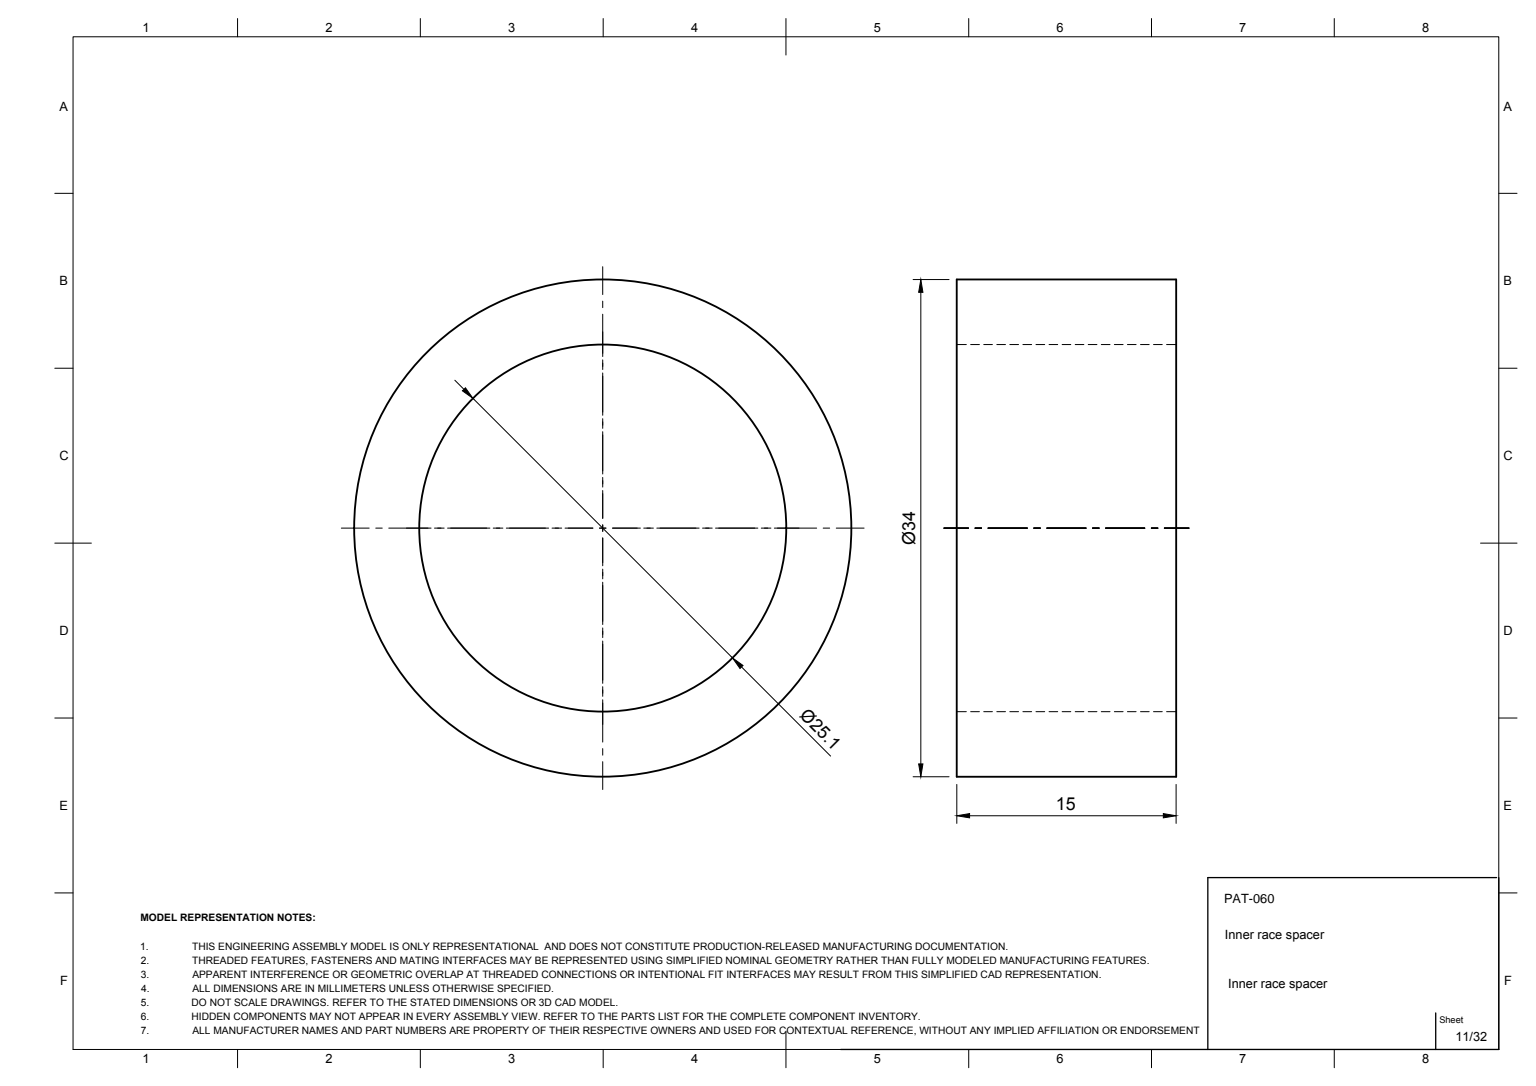
ISO-10303-21;
HEADER;
/* Generated by software containing ST-Developer
 * from STEP Tools, Inc. (www.steptools.com) 
 */

FILE_DESCRIPTION(
/* description */ ('Indexing fixture plate with plunger'),
/* implementation_level */ '2;1');

FILE_NAME(
/* name */ 'Inner race spacer.step',
/* time_stamp */ '2026-10-28T03:23:41-07:00',
/* author */ (''),
/* organization */ (''),
/* preprocessor_version */ 'ST-DEVELOPER v20.2',
/* originating_system */ 'Autodesk Translation Framework v15.17.0.0',
/* authorisation */ '');

FILE_SCHEMA (('AUTOMOTIVE_DESIGN { 1 0 10303 214 3 1 1 }'));
ENDSEC;

DATA;
#10=MECHANICAL_DESIGN_GEOMETRIC_PRESENTATION_REPRESENTATION('',(#323),#10020);
#269=SHAPE_REPRESENTATION_RELATIONSHIP('SRR','None',#10143,#296);
#296=ADVANCED_BREP_SHAPE_REPRESENTATION('',(#359),#9996);
#323=STYLED_ITEM('',(#10368),#359);
#359=MANIFOLD_SOLID_BREP('Body1',#4577);
#412=FACE_BOUND('',#1022,.T.);
#413=FACE_BOUND('',#1024,.T.);
#556=PLANE('',#4998);
#557=PLANE('',#4999);
#708=FACE_OUTER_BOUND('',#1019,.T.);
#709=FACE_OUTER_BOUND('',#1020,.T.);
#710=FACE_OUTER_BOUND('',#1021,.T.);
#711=FACE_OUTER_BOUND('',#1023,.T.);
#1019=EDGE_LOOP('',(#3201,#3202,#3203,#3204));
#1020=EDGE_LOOP('',(#3205,#3206,#3207,#3208));
#1021=EDGE_LOOP('',(#3209));
#1022=EDGE_LOOP('',(#3210));
#1023=EDGE_LOOP('',(#3211));
#1024=EDGE_LOOP('',(#3212));
#1423=LINE('',#7291,#1643);
#1424=LINE('',#7297,#1644);
#1643=VECTOR('',#5778,1.255);
#1644=VECTOR('',#5785,1.7);
#1870=CIRCLE('',#4993,1.255);
#1871=CIRCLE('',#4994,1.255);
#1872=CIRCLE('',#4996,1.7);
#1873=CIRCLE('',#4997,1.7);
#2181=VERTEX_POINT('',#7288);
#2182=VERTEX_POINT('',#7290);
#2183=VERTEX_POINT('',#7294);
#2184=VERTEX_POINT('',#7296);
#2580=EDGE_CURVE('',#2181,#2181,#1870,.T.);
#2581=EDGE_CURVE('',#2181,#2182,#1423,.T.);
#2582=EDGE_CURVE('',#2182,#2182,#1871,.T.);
#2583=EDGE_CURVE('',#2183,#2183,#1872,.T.);
#2584=EDGE_CURVE('',#2183,#2184,#1424,.T.);
#2585=EDGE_CURVE('',#2184,#2184,#1873,.T.);
#3201=ORIENTED_EDGE('',*,*,#2580,.F.);
#3202=ORIENTED_EDGE('',*,*,#2581,.T.);
#3203=ORIENTED_EDGE('',*,*,#2582,.T.);
#3204=ORIENTED_EDGE('',*,*,#2581,.F.);
#3205=ORIENTED_EDGE('',*,*,#2583,.F.);
#3206=ORIENTED_EDGE('',*,*,#2584,.T.);
#3207=ORIENTED_EDGE('',*,*,#2585,.T.);
#3208=ORIENTED_EDGE('',*,*,#2584,.F.);
#3209=ORIENTED_EDGE('',*,*,#2583,.T.);
#3210=ORIENTED_EDGE('',*,*,#2580,.T.);
#3211=ORIENTED_EDGE('',*,*,#2585,.F.);
#3212=ORIENTED_EDGE('',*,*,#2582,.F.);
#4186=CYLINDRICAL_SURFACE('',#4992,1.255);
#4187=CYLINDRICAL_SURFACE('',#4995,1.7);
#4323=ADVANCED_FACE('',(#708),#4186,.F.);
#4324=ADVANCED_FACE('',(#709),#4187,.T.);
#4325=ADVANCED_FACE('',(#710,#412),#556,.T.);
#4326=ADVANCED_FACE('',(#711,#413),#557,.F.);
#4577=CLOSED_SHELL('',(#4323,#4324,#4325,#4326));
#4991=AXIS2_PLACEMENT_3D('',#7286,#5772,#5773);
#4992=AXIS2_PLACEMENT_3D('',#7287,#5774,#5775);
#4993=AXIS2_PLACEMENT_3D('',#7289,#5776,#5777);
#4994=AXIS2_PLACEMENT_3D('',#7292,#5779,#5780);
#4995=AXIS2_PLACEMENT_3D('',#7293,#5781,#5782);
#4996=AXIS2_PLACEMENT_3D('',#7295,#5783,#5784);
#4997=AXIS2_PLACEMENT_3D('',#7298,#5786,#5787);
#4998=AXIS2_PLACEMENT_3D('',#7299,#5788,#5789);
#4999=AXIS2_PLACEMENT_3D('',#7300,#5790,#5791);
#5772=DIRECTION('axis',(0.,0.,1.));
#5773=DIRECTION('refdir',(1.,0.,0.));
#5774=DIRECTION('center_axis',(0.,0.,1.));
#5775=DIRECTION('ref_axis',(1.,0.,0.));
#5776=DIRECTION('center_axis',(0.,0.,-1.));
#5777=DIRECTION('ref_axis',(1.,0.,0.));
#5778=DIRECTION('',(0.,0.,-1.));
#5779=DIRECTION('center_axis',(0.,0.,-1.));
#5780=DIRECTION('ref_axis',(1.,0.,0.));
#5781=DIRECTION('center_axis',(0.,0.,1.));
#5782=DIRECTION('ref_axis',(1.,0.,0.));
#5783=DIRECTION('center_axis',(0.,0.,1.));
#5784=DIRECTION('ref_axis',(1.,0.,0.));
#5785=DIRECTION('',(0.,0.,-1.));
#5786=DIRECTION('center_axis',(0.,0.,1.));
#5787=DIRECTION('ref_axis',(1.,0.,0.));
#5788=DIRECTION('center_axis',(0.,0.,1.));
#5789=DIRECTION('ref_axis',(1.,0.,0.));
#5790=DIRECTION('center_axis',(0.,0.,1.));
#5791=DIRECTION('ref_axis',(1.,0.,0.));
#7286=CARTESIAN_POINT('',(0.,0.,0.));
#7287=CARTESIAN_POINT('Origin',(0.,0.,4.75));
#7288=CARTESIAN_POINT('',(-1.255,-1.53693173292993E-16,6.25));
#7289=CARTESIAN_POINT('Origin',(0.,0.,6.25));
#7290=CARTESIAN_POINT('',(-1.255,-1.53693173292993E-16,4.75));
#7291=CARTESIAN_POINT('',(-1.255,-1.53693173292993E-16,4.75));
#7292=CARTESIAN_POINT('Origin',(0.,0.,4.75));
#7293=CARTESIAN_POINT('Origin',(0.,0.,4.75));
#7294=CARTESIAN_POINT('',(-1.7,-2.0818995585505E-16,6.25));
#7295=CARTESIAN_POINT('Origin',(0.,0.,6.25));
#7296=CARTESIAN_POINT('',(-1.7,-2.0818995585505E-16,4.75));
#7297=CARTESIAN_POINT('',(-1.7,-2.0818995585505E-16,4.75));
#7298=CARTESIAN_POINT('Origin',(0.,0.,4.75));
#7299=CARTESIAN_POINT('Origin',(0.,0.,6.25));
#7300=CARTESIAN_POINT('Origin',(0.,0.,4.75));
#9963=UNCERTAINTY_MEASURE_WITH_UNIT(LENGTH_MEASURE(0.001),#10021,
'DISTANCE_ACCURACY_VALUE',
'Maximum model space distance between geometric entities at asserted c
onnectivities');
#9987=UNCERTAINTY_MEASURE_WITH_UNIT(LENGTH_MEASURE(0.001),#10021,
'DISTANCE_ACCURACY_VALUE',
'Maximum model space distance between geometric entities at asserted c
onnectivities');
#9996=(
GEOMETRIC_REPRESENTATION_CONTEXT(3)
GLOBAL_UNCERTAINTY_ASSIGNED_CONTEXT((#9963))
GLOBAL_UNIT_ASSIGNED_CONTEXT((#10021,#10023,#10024))
REPRESENTATION_CONTEXT('','3D')
);
#10020=(
GEOMETRIC_REPRESENTATION_CONTEXT(3)
GLOBAL_UNCERTAINTY_ASSIGNED_CONTEXT((#9987))
GLOBAL_UNIT_ASSIGNED_CONTEXT((#10021,#10023,#10024))
REPRESENTATION_CONTEXT('','3D')
);
#10021=(
LENGTH_UNIT()
NAMED_UNIT(*)
SI_UNIT(.CENTI.,.METRE.)
);
#10023=(
NAMED_UNIT(*)
PLANE_ANGLE_UNIT()
SI_UNIT($,.RADIAN.)
);
#10024=(
NAMED_UNIT(*)
SI_UNIT($,.STERADIAN.)
SOLID_ANGLE_UNIT()
);
#10033=SHAPE_DEFINITION_REPRESENTATION(#10065,#10143);
#10065=PRODUCT_DEFINITION_SHAPE('',$,#10176);
#10143=SHAPE_REPRESENTATION('',(#4991),#9996);
#10167=PRODUCT_DEFINITION_CONTEXT('part definition',#10265,'design');
#10176=PRODUCT_DEFINITION('Inner race spacer','Inner race spacer',#10208,
#10167);
#10208=PRODUCT_DEFINITION_FORMATION('',$,#10275);
#10265=APPLICATION_CONTEXT(
'Core Data for Automotive Mechanical Design Process');
#10266=PRODUCT_CONTEXT('part definition',#10265,'mechanical');
#10275=PRODUCT('Inner race spacer','Inner race spacer',
'Inner race spacer',(#10266));
#10362=COLOUR_RGB('Grey',0.48,0.52,0.57);
#10363=FILL_AREA_STYLE_COLOUR('',#10362);
#10364=FILL_AREA_STYLE('',(#10363));
#10365=SURFACE_STYLE_FILL_AREA(#10364);
#10366=SURFACE_SIDE_STYLE('',(#10365));
#10367=SURFACE_STYLE_USAGE(.BOTH.,#10366);
#10368=PRESENTATION_STYLE_ASSIGNMENT((#10367));
ENDSEC;
END-ISO-10303-21;
